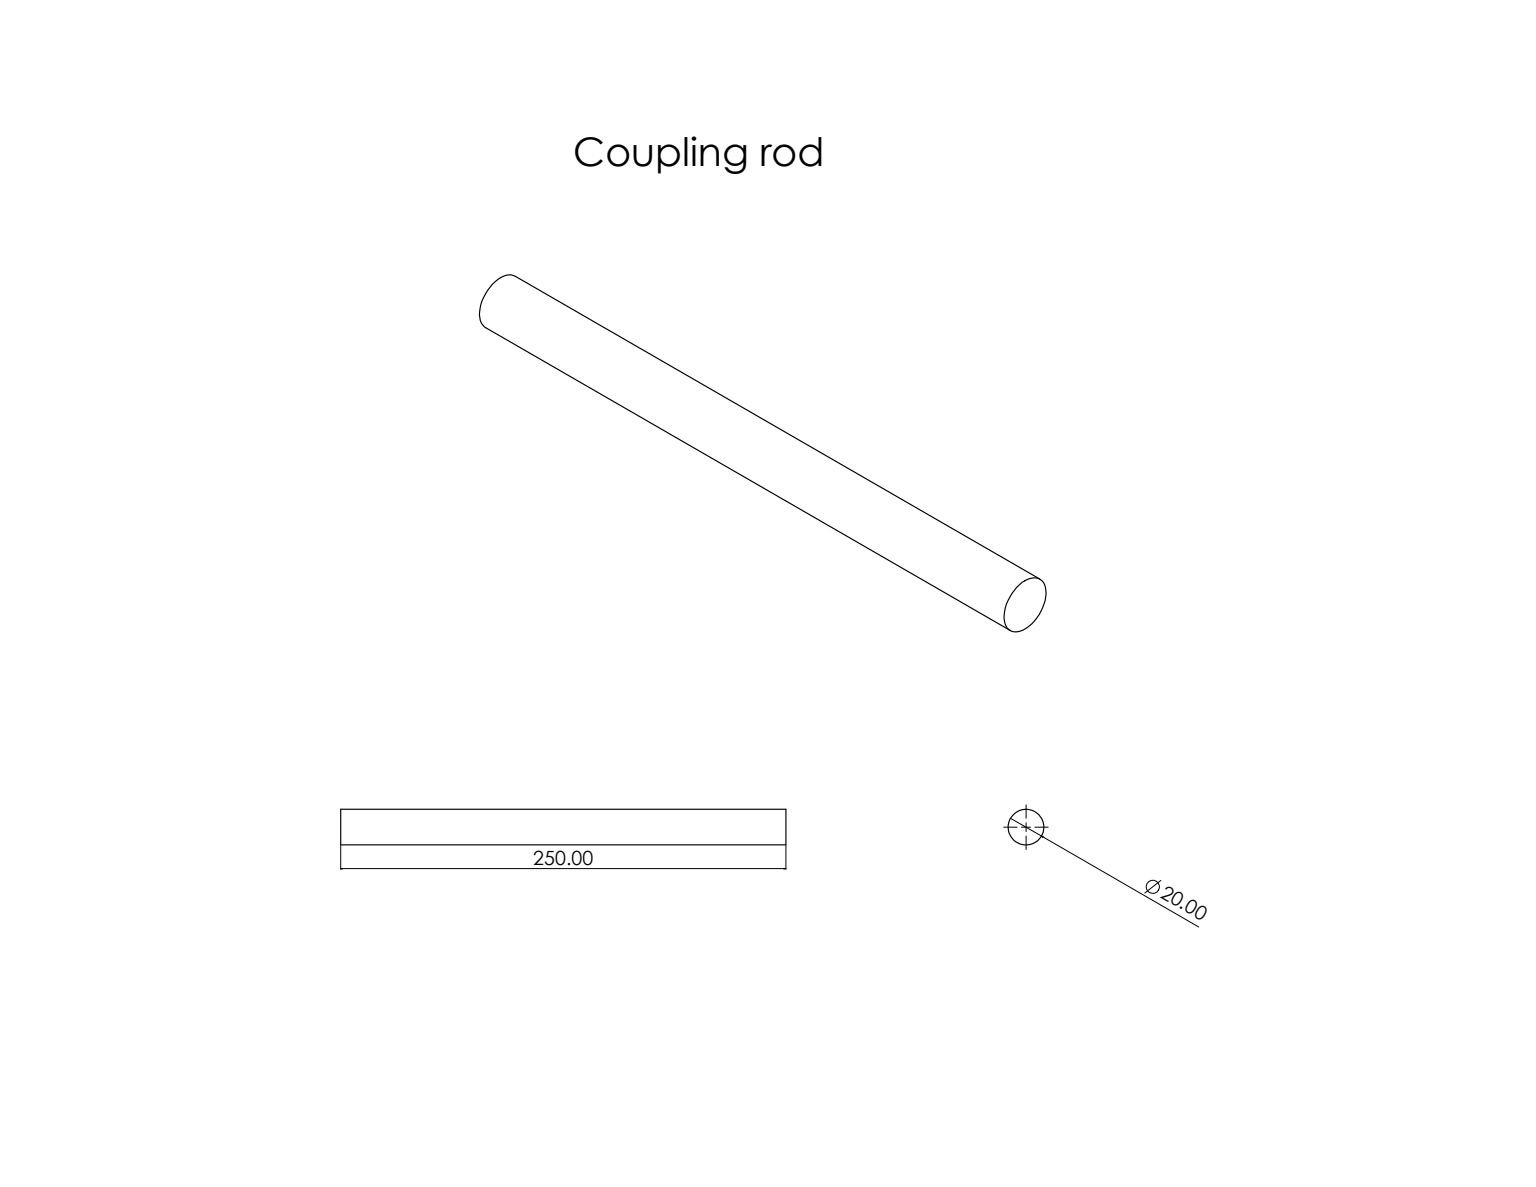
ISO-10303-21;
HEADER;
FILE_DESCRIPTION (('STEP AP214'),
    '1' );
FILE_NAME ('Coupling rod.step',
    '2026-10-27T19:20:31',
    ( '' ),
    ( '' ),
    'SwSTEP 2.0',
    'SolidWorks 2025',
    '' );
FILE_SCHEMA (( 'AUTOMOTIVE_DESIGN' ));
ENDSEC;

DATA;
#22=DIRECTION ( 'NONE',  ( 0.000000000000000000, 0.000000000000000000, 1.000000000000000000 ) ) ;
#296=ORIENTED_EDGE ( 'NONE', *, *, #19861, .T. ) ;
#552=CARTESIAN_POINT ( 'NONE',  ( -362.0709805440841365, 9.999999999999960920, 0.000000000000000000 ) ) ;
#669=CARTESIAN_POINT ( 'NONE',  ( -362.0709805440841365, -10.00000000000005684, 1.224646799147354440E-15 ) ) ;
#690=( NAMED_UNIT ( * ) SI_UNIT ( $, .STERADIAN. ) SOLID_ANGLE_UNIT ( ) );
#951=CARTESIAN_POINT ( 'NONE',  ( -362.0709805440841365, -4.857225732735059864E-14, 0.000000000000000000 ) ) ;
#1246=EDGE_LOOP ( 'NONE', ( #5167, #4784 ) ) ;
#1607=FACE_OUTER_BOUND ( 'NONE', #5363, .T. ) ;
#2038=ORIENTED_EDGE ( 'NONE', *, *, #20881, .F. ) ;
#2090=ORIENTED_EDGE ( 'NONE', *, *, #2687, .T. ) ;
#2358=( GEOMETRIC_REPRESENTATION_CONTEXT ( 3 ) GLOBAL_UNCERTAINTY_ASSIGNED_CONTEXT ( ( #5119 ) ) GLOBAL_UNIT_ASSIGNED_CONTEXT ( ( #23048, #4421, #690 ) ) REPRESENTATION_CONTEXT ( 'NONE', 'WORKASPACE' ) );
#2551=SHAPE_REPRESENTATION_RELATIONSHIP ( 'NONE' , 'NONE' ,  #3691, #22606 ) ;
#2687=EDGE_CURVE ( 'NONE', #18917, #17669, #16627, .T. ) ;
#3119=PRODUCT_DEFINITION_CONTEXT ( 'detailed design', #23780, 'design' ) ;
#3433=AXIS2_PLACEMENT_3D ( 'NONE', #12831, #16813, #20951 ) ;
#3569=PRODUCT_DEFINITION_SHAPE ( 'NONE', 'NONE',  #6229 ) ;
#3591=CARTESIAN_POINT ( 'NONE',  ( -612.0709805440841365, -1.322736627157470569E-16, 0.000000000000000000 ) ) ;
#3592=FACE_OUTER_BOUND ( 'NONE', #26047, .T. ) ;
#3691=SHAPE_REPRESENTATION ( 'Coupling rod', ( #21058 ), #2358 ) ;
#4421=( NAMED_UNIT ( * ) PLANE_ANGLE_UNIT ( ) SI_UNIT ( $, .RADIAN. ) );
#4600=ADVANCED_FACE ( 'NONE', ( #1607 ), #11564, .T. ) ;
#4784=ORIENTED_EDGE ( 'NONE', *, *, #26065, .T. ) ;
#4880=DIRECTION ( 'NONE',  ( 1.000000000000000000, -1.937599346585394162E-16, -0.000000000000000000 ) ) ;
#5029=EDGE_CURVE ( 'NONE', #5443, #17669, #6188, .T. ) ;
#5119=UNCERTAINTY_MEASURE_WITH_UNIT (LENGTH_MEASURE( 1.000000000000000082E-05 ), #23048, 'distance_accuracy_value', 'NONE');
#5167=ORIENTED_EDGE ( 'NONE', *, *, #5029, .T. ) ;
#5363=EDGE_LOOP ( 'NONE', ( #2038, #25045 ) ) ;
#5443=VERTEX_POINT ( 'NONE', #9984 ) ;
#5535=DIRECTION ( 'NONE',  ( 0.000000000000000000, 1.000000000000000000, 0.000000000000000000 ) ) ;
#5819=ADVANCED_FACE ( 'NONE', ( #11118 ), #18842, .T. ) ;
#6188=CIRCLE ( 'NONE', #9578, 10.00000000000004796 ) ;
#6229=PRODUCT_DEFINITION ( 'UNKNOWN', '', #13400, #3119 ) ;
#6811=AXIS2_PLACEMENT_3D ( 'NONE', #25173, #24906, #8931 ) ;
#6847=AXIS2_PLACEMENT_3D ( 'NONE', #3591, #9845, #19089 ) ;
#7873=MECHANICAL_DESIGN_GEOMETRIC_PRESENTATION_REPRESENTATION('',(#16380),#24910);
#7994=CARTESIAN_POINT ( 'NONE',  ( 0.000000000000000000, 0.000000000000000000, 0.000000000000000000 ) ) ;
#8012=DIRECTION ( 'NONE',  ( 1.000000000000000000, -1.937599346585394162E-16, -0.000000000000000000 ) ) ;
#8436=AXIS2_PLACEMENT_3D ( 'NONE', #9712, #13443, #19559 ) ;
#8645=DIRECTION ( 'NONE',  ( 1.000000000000000000, -1.937599346585394162E-16, -0.000000000000000000 ) ) ;
#8656=LINE ( 'NONE', #552, #13462 ) ;
#8833=ORIENTED_EDGE ( 'NONE', *, *, #5029, .F. ) ;
#8931=DIRECTION ( 'NONE',  ( 0.000000000000000000, 1.000000000000000000, 0.000000000000000000 ) ) ;
#8975=MANIFOLD_SOLID_BREP ( 'Revolve3', #18975 ) ;
#9059=DIRECTION ( 'NONE',  ( 1.000000000000000000, -1.937599346585394162E-16, -0.000000000000000000 ) ) ;
#9115=CARTESIAN_POINT ( 'NONE',  ( -362.0709805440841365, -4.857225732735059864E-14, 0.000000000000000000 ) ) ;
#9398=CARTESIAN_POINT ( 'NONE',  ( -612.0709805440841365, -1.322736627157445917E-16, 0.000000000000000000 ) ) ;
#9466=ORIENTED_EDGE ( 'NONE', *, *, #26065, .F. ) ;
#9578=AXIS2_PLACEMENT_3D ( 'NONE', #20131, #8012, #23847 ) ;
#9712=CARTESIAN_POINT ( 'NONE',  ( -362.0709805440841365, -4.857225732735059864E-14, 0.000000000000000000 ) ) ;
#9845=DIRECTION ( 'NONE',  ( -1.000000000000000000, 1.937599346585394162E-16, 0.000000000000000000 ) ) ;
#9984=CARTESIAN_POINT ( 'NONE',  ( -362.0709805440841365, 10.00000000000000000, 0.000000000000000000 ) ) ;
#10633=ADVANCED_FACE ( 'NONE', ( #3592 ), #23810, .T. ) ;
#10660=DIRECTION ( 'NONE',  ( 1.937599346585394162E-16, 1.000000000000000000, 0.000000000000000000 ) ) ;
#11055=FACE_OUTER_BOUND ( 'NONE', #1246, .T. ) ;
#11118=FACE_OUTER_BOUND ( 'NONE', #16211, .T. ) ;
#11564=PLANE ( 'NONE',  #6847 ) ;
#12831=CARTESIAN_POINT ( 'NONE',  ( -612.0709805440841365, -1.322736627157445917E-16, 0.000000000000000000 ) ) ;
#13400=PRODUCT_DEFINITION_FORMATION_WITH_SPECIFIED_SOURCE ( 'ANY', '', #13756, .NOT_KNOWN. ) ;
#13443=DIRECTION ( 'NONE',  ( 1.000000000000000000, -1.937599346585394162E-16, -0.000000000000000000 ) ) ;
#13462=VECTOR ( 'NONE', #19415, 1000.000000000000000 ) ;
#13756=PRODUCT ( 'Coupling rod', 'Coupling rod', '', ( #25945 ) ) ;
#13943=SHAPE_DEFINITION_REPRESENTATION ( #3569, #3691 ) ;
#14068=CIRCLE ( 'NONE', #14917, 9.999999999999969802 ) ;
#14917=AXIS2_PLACEMENT_3D ( 'NONE', #9398, #17628, #5535 ) ;
#14974=DIRECTION ( 'NONE',  ( 0.000000000000000000, 1.000000000000000000, 0.000000000000000000 ) ) ;
#15144=EDGE_CURVE ( 'NONE', #19457, #5443, #8656, .T. ) ;
#15977=DIRECTION ( 'NONE',  ( 1.000000000000000000, 0.000000000000000000, 0.000000000000000000 ) ) ;
#16211=EDGE_LOOP ( 'NONE', ( #22780, #2090, #8833, #20519 ) ) ;
#16380=STYLED_ITEM('',(#26395),#8975);
#16627=LINE ( 'NONE', #669, #23612 ) ;
#16813=DIRECTION ( 'NONE',  ( 1.000000000000000000, -1.937599346585394162E-16, -0.000000000000000000 ) ) ;
#17628=DIRECTION ( 'NONE',  ( 1.000000000000000000, -1.937599346585394162E-16, -0.000000000000000000 ) ) ;
#17669=VERTEX_POINT ( 'NONE', #18856 ) ;
#18842=CYLINDRICAL_SURFACE ( 'NONE', #24040, 10.00000000000000888 ) ;
#18856=CARTESIAN_POINT ( 'NONE',  ( -362.0709805440841365, -10.00000000000009770, 1.224646799147362328E-15 ) ) ;
#18917=VERTEX_POINT ( 'NONE', #26050 ) ;
#18975=CLOSED_SHELL ( 'NONE', ( #5819, #4600, #10633, #24792 ) ) ;
#19089=DIRECTION ( 'NONE',  ( -1.937599346585394162E-16, -1.000000000000000000, 0.000000000000000000 ) ) ;
#19167=PLANE ( 'NONE',  #19520 ) ;
#19262=ORIENTED_EDGE ( 'NONE', *, *, #2687, .F. ) ;
#19415=DIRECTION ( 'NONE',  ( 1.000000000000000000, -1.937599346585394162E-16, -0.000000000000000000 ) ) ;
#19457=VERTEX_POINT ( 'NONE', #23204 ) ;
#19520=AXIS2_PLACEMENT_3D ( 'NONE', #951, #9059, #10660 ) ;
#19559=DIRECTION ( 'NONE',  ( 0.000000000000000000, 1.000000000000000000, 0.000000000000000000 ) ) ;
#19861=EDGE_CURVE ( 'NONE', #18917, #19457, #25988, .T. ) ;
#20131=CARTESIAN_POINT ( 'NONE',  ( -362.0709805440841365, -4.857225732735059864E-14, 0.000000000000000000 ) ) ;
#20397=( NAMED_UNIT ( * ) PLANE_ANGLE_UNIT ( ) SI_UNIT ( $, .RADIAN. ) );
#20471=APPLICATION_CONTEXT ( 'automotive_design' ) ;
#20519=ORIENTED_EDGE ( 'NONE', *, *, #15144, .F. ) ;
#20881=EDGE_CURVE ( 'NONE', #19457, #18917, #14068, .T. ) ;
#20951=DIRECTION ( 'NONE',  ( 0.000000000000000000, 1.000000000000000000, 0.000000000000000000 ) ) ;
#21058=AXIS2_PLACEMENT_3D ( 'NONE', #7994, #22, #15977 ) ;
#22264=( LENGTH_UNIT ( ) NAMED_UNIT ( * ) SI_UNIT ( .MILLI., .METRE. ) );
#22606=ADVANCED_BREP_SHAPE_REPRESENTATION ( '', ( #8975, #21058 ), #2358 ) ;
#22780=ORIENTED_EDGE ( 'NONE', *, *, #20881, .T. ) ;
#22967=CIRCLE ( 'NONE', #6811, 10.00000000000004796 ) ;
#23048=( LENGTH_UNIT ( ) NAMED_UNIT ( * ) SI_UNIT ( .MILLI., .METRE. ) );
#23204=CARTESIAN_POINT ( 'NONE',  ( -612.0709805440841365, 9.999999999999969802, 0.000000000000000000 ) ) ;
#23425=ORIENTED_EDGE ( 'NONE', *, *, #15144, .T. ) ;
#23612=VECTOR ( 'NONE', #8645, 1000.000000000000000 ) ;
#23780=APPLICATION_CONTEXT ( 'automotive_design' ) ;
#23810=CYLINDRICAL_SURFACE ( 'NONE', #8436, 10.00000000000000888 ) ;
#23847=DIRECTION ( 'NONE',  ( 0.000000000000000000, 1.000000000000000000, 0.000000000000000000 ) ) ;
#24040=AXIS2_PLACEMENT_3D ( 'NONE', #9115, #4880, #14974 ) ;
#24253=( NAMED_UNIT ( * ) SI_UNIT ( $, .STERADIAN. ) SOLID_ANGLE_UNIT ( ) );
#24294=UNCERTAINTY_MEASURE_WITH_UNIT (LENGTH_MEASURE( 1.000000000000000082E-05 ), #22264, 'distance_accuracy_value', 'NONE');
#24792=ADVANCED_FACE ( 'NONE', ( #11055 ), #19167, .T. ) ;
#24906=DIRECTION ( 'NONE',  ( 1.000000000000000000, -1.937599346585394162E-16, -0.000000000000000000 ) ) ;
#24910=( GEOMETRIC_REPRESENTATION_CONTEXT ( 3 ) GLOBAL_UNCERTAINTY_ASSIGNED_CONTEXT ( ( #24294 ) ) GLOBAL_UNIT_ASSIGNED_CONTEXT ( ( #22264, #20397, #24253 ) ) REPRESENTATION_CONTEXT ( 'NONE', 'WORKASPACE' ) );
#25045=ORIENTED_EDGE ( 'NONE', *, *, #19861, .F. ) ;
#25173=CARTESIAN_POINT ( 'NONE',  ( -362.0709805440841365, -4.857225732735059864E-14, 0.000000000000000000 ) ) ;
#25945=PRODUCT_CONTEXT ( 'NONE', #20471, 'mechanical' ) ;
#25988=CIRCLE ( 'NONE', #3433, 9.999999999999969802 ) ;
#26047=EDGE_LOOP ( 'NONE', ( #19262, #296, #23425, #9466 ) ) ;
#26050=CARTESIAN_POINT ( 'NONE',  ( -612.0709805440841365, -9.999999999999969802, 1.224646799147352073E-15 ) ) ;
#26065=EDGE_CURVE ( 'NONE', #17669, #5443, #22967, .T. ) ;
#26389=COLOUR_RGB('Grey',0.48,0.52,0.57);
#26390=FILL_AREA_STYLE_COLOUR('',#26389);
#26391=FILL_AREA_STYLE('',(#26390));
#26392=SURFACE_STYLE_FILL_AREA(#26391);
#26393=SURFACE_SIDE_STYLE('',(#26392));
#26394=SURFACE_STYLE_USAGE(.BOTH.,#26393);
#26395=PRESENTATION_STYLE_ASSIGNMENT((#26394));
ENDSEC;
END-ISO-10303-21;
